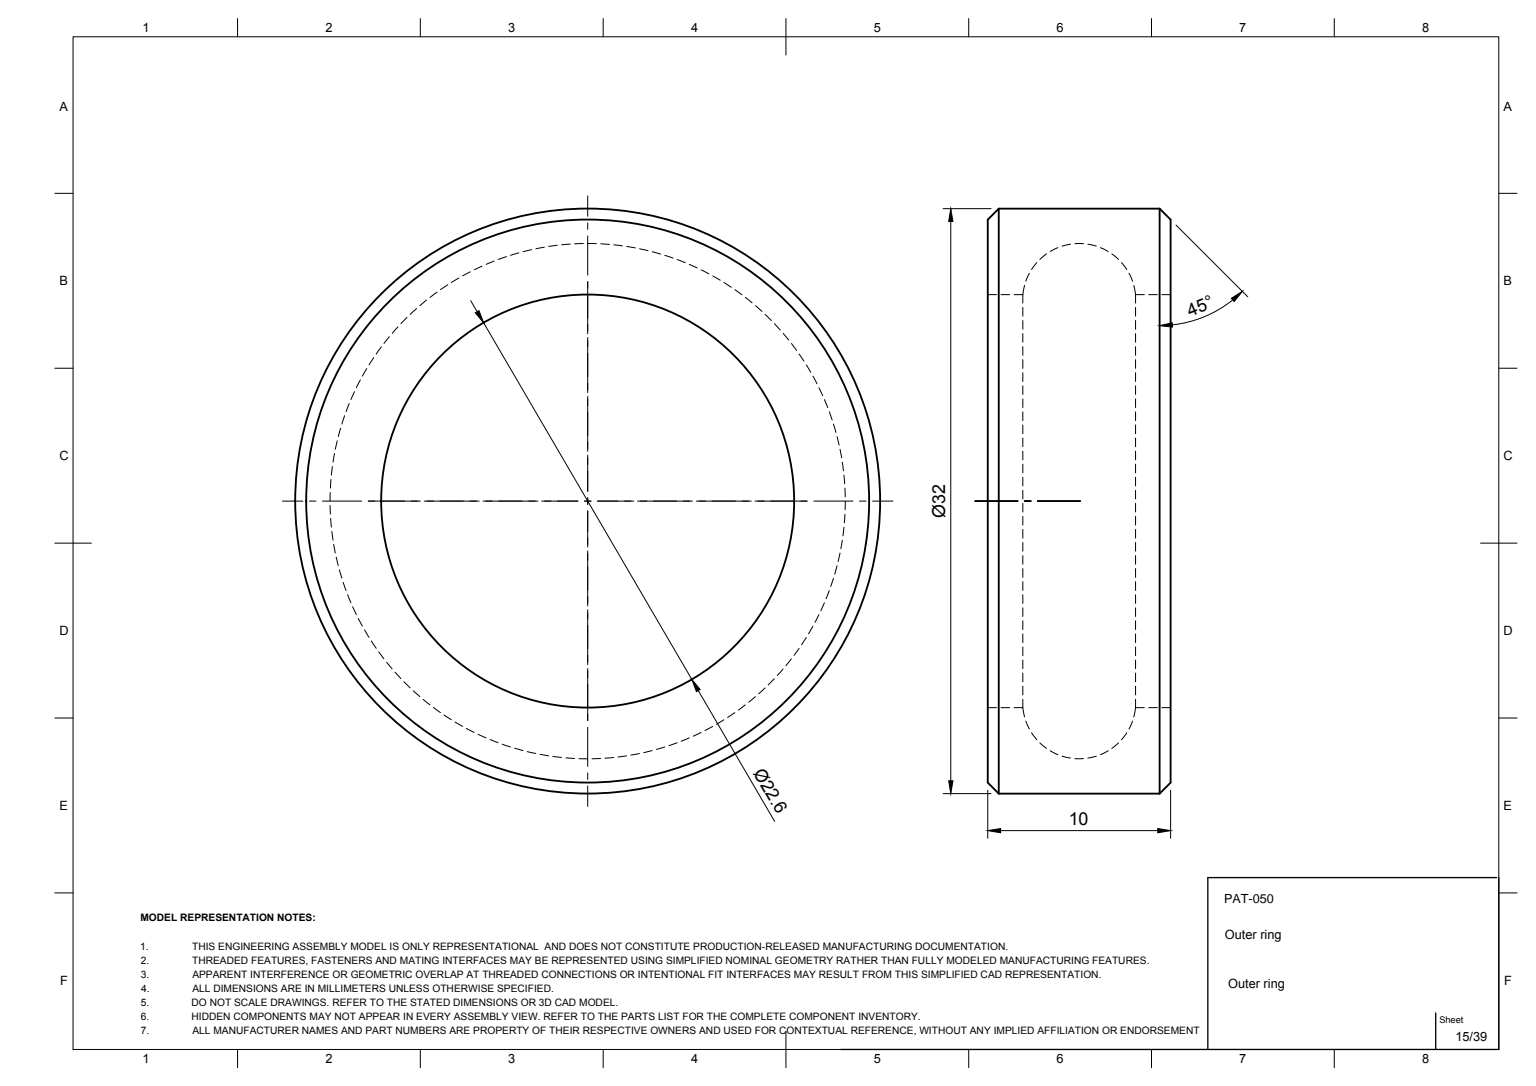
ISO-10303-21;
HEADER;
/* Generated by software containing ST-Developer
 * from STEP Tools, Inc. (www.steptools.com) 
 */

FILE_DESCRIPTION(
/* description */ ('Hand wheel with handle and shaft collar'),
/* implementation_level */ '2;1');

FILE_NAME(
/* name */ 'Outer ring.step',
/* time_stamp */ '2026-10-28T03:23:19-07:00',
/* author */ (''),
/* organization */ (''),
/* preprocessor_version */ 'ST-DEVELOPER v20.2',
/* originating_system */ 'Autodesk Translation Framework v15.17.0.0',
/* authorisation */ '');

FILE_SCHEMA (('AUTOMOTIVE_DESIGN { 1 0 10303 214 3 1 1 }'));
ENDSEC;

DATA;
#10=MECHANICAL_DESIGN_GEOMETRIC_PRESENTATION_REPRESENTATION('',(#405),#10510);
#298=TOROIDAL_SURFACE('',#5884,1.1,0.309556);
#306=CONICAL_SURFACE('',#5895,1.57,0.785398163397449);
#307=CONICAL_SURFACE('',#5899,1.57,0.785398163397449);
#341=SHAPE_REPRESENTATION_RELATIONSHIP('SRR','None',#10658,#373);
#373=ADVANCED_BREP_SHAPE_REPRESENTATION('',(#451),#10485);
#405=STYLED_ITEM('',(#10908),#451);
#451=MANIFOLD_SOLID_BREP('Body1',#5305);
#541=FACE_BOUND('',#1233,.T.);
#542=FACE_BOUND('',#1238,.T.);
#649=PLANE('',#5892);
#650=PLANE('',#5901);
#856=FACE_OUTER_BOUND('',#1230,.T.);
#857=FACE_OUTER_BOUND('',#1231,.T.);
#858=FACE_OUTER_BOUND('',#1232,.T.);
#859=FACE_OUTER_BOUND('',#1234,.T.);
#860=FACE_OUTER_BOUND('',#1235,.T.);
#861=FACE_OUTER_BOUND('',#1236,.T.);
#862=FACE_OUTER_BOUND('',#1237,.T.);
#863=FACE_OUTER_BOUND('',#1239,.T.);
#1230=EDGE_LOOP('',(#3955,#3956,#3957,#3958,#3959,#3960));
#1231=EDGE_LOOP('',(#3961,#3962,#3963,#3964,#3965));
#1232=EDGE_LOOP('',(#3966));
#1233=EDGE_LOOP('',(#3967));
#1234=EDGE_LOOP('',(#3968,#3969,#3970,#3971));
#1235=EDGE_LOOP('',(#3972,#3973,#3974,#3975));
#1236=EDGE_LOOP('',(#3976,#3977,#3978,#3979));
#1237=EDGE_LOOP('',(#3980));
#1238=EDGE_LOOP('',(#3981));
#1239=EDGE_LOOP('',(#3982,#3983,#3984,#3985,#3986));
#1632=LINE('',#8623,#1942);
#1633=LINE('',#8632,#1943);
#1634=LINE('',#8636,#1944);
#1635=LINE('',#8640,#1945);
#1636=LINE('',#8643,#1946);
#1942=VECTOR('',#6928,1.129765);
#1943=VECTOR('',#6939,1.57);
#1944=VECTOR('',#6944,1.6);
#1945=VECTOR('',#6949,1.57);
#1946=VECTOR('',#6954,1.129765);
#2213=CIRCLE('',#5885,1.129765);
#2214=CIRCLE('',#5886,1.129765);
#2215=CIRCLE('',#5887,0.309556);
#2216=CIRCLE('',#5888,1.129765);
#2217=CIRCLE('',#5889,1.129765);
#2218=CIRCLE('',#5891,1.129765);
#2219=CIRCLE('',#5893,1.54);
#2220=CIRCLE('',#5894,1.129765);
#2221=CIRCLE('',#5896,1.6);
#2222=CIRCLE('',#5898,1.6);
#2223=CIRCLE('',#5900,1.54);
#2575=VERTEX_POINT('',#8611);
#2576=VERTEX_POINT('',#8612);
#2577=VERTEX_POINT('',#8615);
#2578=VERTEX_POINT('',#8617);
#2579=VERTEX_POINT('',#8621);
#2580=VERTEX_POINT('',#8625);
#2581=VERTEX_POINT('',#8627);
#2582=VERTEX_POINT('',#8630);
#2583=VERTEX_POINT('',#8634);
#2584=VERTEX_POINT('',#8638);
#3095=EDGE_CURVE('',#2575,#2576,#2213,.T.);
#3096=EDGE_CURVE('',#2576,#2575,#2214,.T.);
#3097=EDGE_CURVE('',#2576,#2577,#2215,.T.);
#3098=EDGE_CURVE('',#2578,#2577,#2216,.T.);
#3099=EDGE_CURVE('',#2577,#2578,#2217,.T.);
#3100=EDGE_CURVE('',#2579,#2579,#2218,.T.);
#3101=EDGE_CURVE('',#2579,#2578,#1632,.T.);
#3102=EDGE_CURVE('',#2580,#2580,#2219,.T.);
#3103=EDGE_CURVE('',#2581,#2581,#2220,.T.);
#3104=EDGE_CURVE('',#2582,#2582,#2221,.T.);
#3105=EDGE_CURVE('',#2582,#2580,#1633,.T.);
#3106=EDGE_CURVE('',#2583,#2583,#2222,.T.);
#3107=EDGE_CURVE('',#2583,#2582,#1634,.T.);
#3108=EDGE_CURVE('',#2584,#2584,#2223,.T.);
#3109=EDGE_CURVE('',#2584,#2583,#1635,.T.);
#3110=EDGE_CURVE('',#2575,#2581,#1636,.T.);
#3955=ORIENTED_EDGE('',*,*,#3095,.F.);
#3956=ORIENTED_EDGE('',*,*,#3096,.F.);
#3957=ORIENTED_EDGE('',*,*,#3097,.T.);
#3958=ORIENTED_EDGE('',*,*,#3098,.F.);
#3959=ORIENTED_EDGE('',*,*,#3099,.F.);
#3960=ORIENTED_EDGE('',*,*,#3097,.F.);
#3961=ORIENTED_EDGE('',*,*,#3100,.T.);
#3962=ORIENTED_EDGE('',*,*,#3101,.T.);
#3963=ORIENTED_EDGE('',*,*,#3098,.T.);
#3964=ORIENTED_EDGE('',*,*,#3099,.T.);
#3965=ORIENTED_EDGE('',*,*,#3101,.F.);
#3966=ORIENTED_EDGE('',*,*,#3102,.F.);
#3967=ORIENTED_EDGE('',*,*,#3103,.T.);
#3968=ORIENTED_EDGE('',*,*,#3104,.F.);
#3969=ORIENTED_EDGE('',*,*,#3105,.T.);
#3970=ORIENTED_EDGE('',*,*,#3102,.T.);
#3971=ORIENTED_EDGE('',*,*,#3105,.F.);
#3972=ORIENTED_EDGE('',*,*,#3106,.F.);
#3973=ORIENTED_EDGE('',*,*,#3107,.T.);
#3974=ORIENTED_EDGE('',*,*,#3104,.T.);
#3975=ORIENTED_EDGE('',*,*,#3107,.F.);
#3976=ORIENTED_EDGE('',*,*,#3108,.F.);
#3977=ORIENTED_EDGE('',*,*,#3109,.T.);
#3978=ORIENTED_EDGE('',*,*,#3106,.T.);
#3979=ORIENTED_EDGE('',*,*,#3109,.F.);
#3980=ORIENTED_EDGE('',*,*,#3108,.T.);
#3981=ORIENTED_EDGE('',*,*,#3100,.F.);
#3982=ORIENTED_EDGE('',*,*,#3095,.T.);
#3983=ORIENTED_EDGE('',*,*,#3096,.T.);
#3984=ORIENTED_EDGE('',*,*,#3110,.T.);
#3985=ORIENTED_EDGE('',*,*,#3103,.F.);
#3986=ORIENTED_EDGE('',*,*,#3110,.F.);
#4915=CYLINDRICAL_SURFACE('',#5890,1.129765);
#4916=CYLINDRICAL_SURFACE('',#5897,1.6);
#4917=CYLINDRICAL_SURFACE('',#5902,1.129765);
#5068=ADVANCED_FACE('',(#856),#298,.F.);
#5069=ADVANCED_FACE('',(#857),#4915,.F.);
#5070=ADVANCED_FACE('',(#858,#541),#649,.T.);
#5071=ADVANCED_FACE('',(#859),#306,.T.);
#5072=ADVANCED_FACE('',(#860),#4916,.T.);
#5073=ADVANCED_FACE('',(#861),#307,.T.);
#5074=ADVANCED_FACE('',(#862,#542),#650,.T.);
#5075=ADVANCED_FACE('',(#863),#4917,.F.);
#5305=CLOSED_SHELL('',(#5068,#5069,#5070,#5071,#5072,#5073,#5074,#5075));
#5883=AXIS2_PLACEMENT_3D('',#8609,#6910,#6911);
#5884=AXIS2_PLACEMENT_3D('',#8610,#6912,#6913);
#5885=AXIS2_PLACEMENT_3D('',#8613,#6914,#6915);
#5886=AXIS2_PLACEMENT_3D('',#8614,#6916,#6917);
#5887=AXIS2_PLACEMENT_3D('',#8616,#6918,#6919);
#5888=AXIS2_PLACEMENT_3D('',#8618,#6920,#6921);
#5889=AXIS2_PLACEMENT_3D('',#8619,#6922,#6923);
#5890=AXIS2_PLACEMENT_3D('',#8620,#6924,#6925);
#5891=AXIS2_PLACEMENT_3D('',#8622,#6926,#6927);
#5892=AXIS2_PLACEMENT_3D('',#8624,#6929,#6930);
#5893=AXIS2_PLACEMENT_3D('',#8626,#6931,#6932);
#5894=AXIS2_PLACEMENT_3D('',#8628,#6933,#6934);
#5895=AXIS2_PLACEMENT_3D('',#8629,#6935,#6936);
#5896=AXIS2_PLACEMENT_3D('',#8631,#6937,#6938);
#5897=AXIS2_PLACEMENT_3D('',#8633,#6940,#6941);
#5898=AXIS2_PLACEMENT_3D('',#8635,#6942,#6943);
#5899=AXIS2_PLACEMENT_3D('',#8637,#6945,#6946);
#5900=AXIS2_PLACEMENT_3D('',#8639,#6947,#6948);
#5901=AXIS2_PLACEMENT_3D('',#8641,#6950,#6951);
#5902=AXIS2_PLACEMENT_3D('',#8642,#6952,#6953);
#6910=DIRECTION('axis',(0.,0.,1.));
#6911=DIRECTION('refdir',(1.,0.,0.));
#6912=DIRECTION('center_axis',(0.,-1.,0.));
#6913=DIRECTION('ref_axis',(0.,0.,-1.));
#6914=DIRECTION('center_axis',(0.,-1.,0.));
#6915=DIRECTION('ref_axis',(1.,0.,0.));
#6916=DIRECTION('center_axis',(0.,-1.,0.));
#6917=DIRECTION('ref_axis',(1.,0.,0.));
#6918=DIRECTION('center_axis',(1.,0.,1.22464679914735E-16));
#6919=DIRECTION('ref_axis',(-1.22464679914735E-16,0.,1.));
#6920=DIRECTION('center_axis',(0.,1.,0.));
#6921=DIRECTION('ref_axis',(1.,0.,0.));
#6922=DIRECTION('center_axis',(0.,1.,0.));
#6923=DIRECTION('ref_axis',(1.,0.,0.));
#6924=DIRECTION('center_axis',(0.,-1.,0.));
#6925=DIRECTION('ref_axis',(1.,0.,0.));
#6926=DIRECTION('center_axis',(0.,-1.,0.));
#6927=DIRECTION('ref_axis',(1.,0.,0.));
#6928=DIRECTION('',(0.,1.,0.));
#6929=DIRECTION('center_axis',(0.,1.,0.));
#6930=DIRECTION('ref_axis',(0.,0.,1.));
#6931=DIRECTION('center_axis',(0.,-1.,0.));
#6932=DIRECTION('ref_axis',(1.,0.,0.));
#6933=DIRECTION('center_axis',(0.,-1.,0.));
#6934=DIRECTION('ref_axis',(1.,0.,0.));
#6935=DIRECTION('center_axis',(0.,-1.,0.));
#6936=DIRECTION('ref_axis',(1.,0.,0.));
#6937=DIRECTION('center_axis',(0.,-1.,0.));
#6938=DIRECTION('ref_axis',(1.,0.,0.));
#6939=DIRECTION('',(0.707106781186548,0.707106781186547,8.65956056235494E-17));
#6940=DIRECTION('center_axis',(0.,-1.,0.));
#6941=DIRECTION('ref_axis',(1.,0.,0.));
#6942=DIRECTION('center_axis',(0.,-1.,0.));
#6943=DIRECTION('ref_axis',(1.,0.,0.));
#6944=DIRECTION('',(0.,1.,0.));
#6945=DIRECTION('center_axis',(0.,1.,0.));
#6946=DIRECTION('ref_axis',(1.,0.,0.));
#6947=DIRECTION('center_axis',(0.,-1.,0.));
#6948=DIRECTION('ref_axis',(1.,0.,0.));
#6949=DIRECTION('',(-0.707106781186548,0.707106781186547,-8.65956056235494E-17));
#6950=DIRECTION('center_axis',(0.,-1.,0.));
#6951=DIRECTION('ref_axis',(0.,0.,-1.));
#6952=DIRECTION('center_axis',(0.,-1.,0.));
#6953=DIRECTION('ref_axis',(1.,0.,0.));
#6954=DIRECTION('',(0.,1.,0.));
#8609=CARTESIAN_POINT('',(0.,0.,0.));
#8610=CARTESIAN_POINT('Origin',(0.,0.,0.));
#8611=CARTESIAN_POINT('',(-1.129765,0.308121667383195,-1.38356309103871E-16));
#8612=CARTESIAN_POINT('',(-1.38356309103871E-16,0.308121667383195,1.129765));
#8613=CARTESIAN_POINT('Origin',(0.,0.308121667383195,0.));
#8614=CARTESIAN_POINT('Origin',(0.,0.308121667383195,0.));
#8615=CARTESIAN_POINT('',(-1.38356309103871E-16,-0.308121667383195,1.129765));
#8616=CARTESIAN_POINT('Origin',(-1.34711147906209E-16,0.,1.1));
#8617=CARTESIAN_POINT('',(-1.129765,-0.308121667383195,1.38356309103871E-16));
#8618=CARTESIAN_POINT('Origin',(0.,-0.308121667383195,0.));
#8619=CARTESIAN_POINT('Origin',(0.,-0.308121667383195,0.));
#8620=CARTESIAN_POINT('Origin',(0.,0.,0.));
#8621=CARTESIAN_POINT('',(-1.129765,-0.5,-1.38356309103871E-16));
#8622=CARTESIAN_POINT('Origin',(0.,-0.5,0.));
#8623=CARTESIAN_POINT('',(-1.129765,0.,-1.38356309103871E-16));
#8624=CARTESIAN_POINT('Origin',(1.54,0.5,0.));
#8625=CARTESIAN_POINT('',(-1.54,0.5,-1.88595607068692E-16));
#8626=CARTESIAN_POINT('Origin',(0.,0.5,0.));
#8627=CARTESIAN_POINT('',(-1.129765,0.5,-1.38356309103871E-16));
#8628=CARTESIAN_POINT('Origin',(0.,0.5,0.));
#8629=CARTESIAN_POINT('Origin',(0.,0.47,0.));
#8630=CARTESIAN_POINT('',(-1.6,0.44,-1.95943487863577E-16));
#8631=CARTESIAN_POINT('Origin',(0.,0.44,0.));
#8632=CARTESIAN_POINT('',(-1.57,0.47,-1.92269547466134E-16));
#8633=CARTESIAN_POINT('Origin',(0.,0.,0.));
#8634=CARTESIAN_POINT('',(-1.6,-0.44,-1.95943487863577E-16));
#8635=CARTESIAN_POINT('Origin',(0.,-0.44,0.));
#8636=CARTESIAN_POINT('',(-1.6,0.,-1.95943487863577E-16));
#8637=CARTESIAN_POINT('Origin',(0.,-0.47,0.));
#8638=CARTESIAN_POINT('',(-1.54,-0.5,-1.88595607068692E-16));
#8639=CARTESIAN_POINT('Origin',(0.,-0.5,0.));
#8640=CARTESIAN_POINT('',(-1.57,-0.47,-1.92269547466134E-16));
#8641=CARTESIAN_POINT('Origin',(1.129765,-0.5,0.));
#8642=CARTESIAN_POINT('Origin',(0.,0.,0.));
#8643=CARTESIAN_POINT('',(-1.129765,0.,-1.38356309103871E-16));
#10446=UNCERTAINTY_MEASURE_WITH_UNIT(LENGTH_MEASURE(0.001),#10511,
'DISTANCE_ACCURACY_VALUE',
'Maximum model space distance between geometric entities at asserted c
onnectivities');
#10471=UNCERTAINTY_MEASURE_WITH_UNIT(LENGTH_MEASURE(0.001),#10511,
'DISTANCE_ACCURACY_VALUE',
'Maximum model space distance between geometric entities at asserted c
onnectivities');
#10485=(
GEOMETRIC_REPRESENTATION_CONTEXT(3)
GLOBAL_UNCERTAINTY_ASSIGNED_CONTEXT((#10446))
GLOBAL_UNIT_ASSIGNED_CONTEXT((#10511,#10513,#10514))
REPRESENTATION_CONTEXT('','3D')
);
#10510=(
GEOMETRIC_REPRESENTATION_CONTEXT(3)
GLOBAL_UNCERTAINTY_ASSIGNED_CONTEXT((#10471))
GLOBAL_UNIT_ASSIGNED_CONTEXT((#10511,#10513,#10514))
REPRESENTATION_CONTEXT('','3D')
);
#10511=(
LENGTH_UNIT()
NAMED_UNIT(*)
SI_UNIT(.CENTI.,.METRE.)
);
#10513=(
NAMED_UNIT(*)
PLANE_ANGLE_UNIT()
SI_UNIT($,.RADIAN.)
);
#10514=(
NAMED_UNIT(*)
SI_UNIT($,.STERADIAN.)
SOLID_ANGLE_UNIT()
);
#10528=SHAPE_DEFINITION_REPRESENTATION(#10566,#10658);
#10566=PRODUCT_DEFINITION_SHAPE('',$,#10697);
#10658=SHAPE_REPRESENTATION('',(#5883),#10485);
#10683=PRODUCT_DEFINITION_CONTEXT('part definition',#10799,'design');
#10697=PRODUCT_DEFINITION('Outer ring','Outer ring',#10735,#10683);
#10735=PRODUCT_DEFINITION_FORMATION('',$,#10814);
#10799=APPLICATION_CONTEXT(
'Core Data for Automotive Mechanical Design Process');
#10800=PRODUCT_CONTEXT('part definition',#10799,'mechanical');
#10814=PRODUCT('Outer ring','Outer ring','Outer ring',(#10800));
#10902=COLOUR_RGB('Grey',0.48,0.52,0.57);
#10903=FILL_AREA_STYLE_COLOUR('',#10902);
#10904=FILL_AREA_STYLE('',(#10903));
#10905=SURFACE_STYLE_FILL_AREA(#10904);
#10906=SURFACE_SIDE_STYLE('',(#10905));
#10907=SURFACE_STYLE_USAGE(.BOTH.,#10906);
#10908=PRESENTATION_STYLE_ASSIGNMENT((#10907));
ENDSEC;
END-ISO-10303-21;
